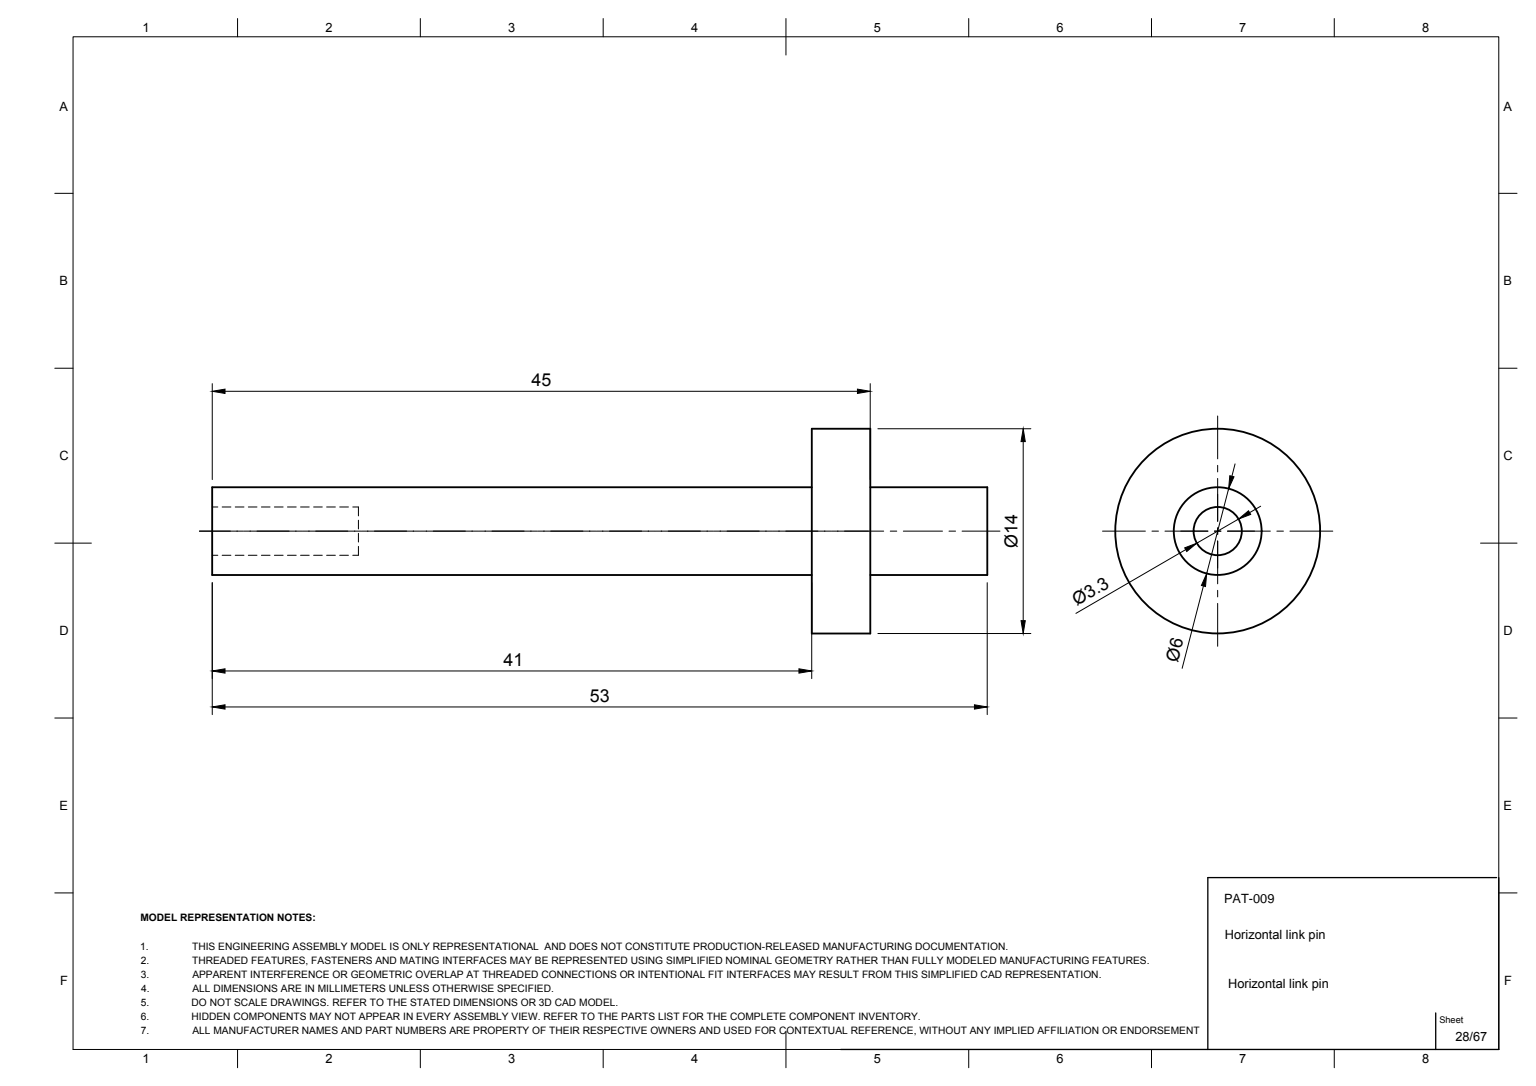
ISO-10303-21;
HEADER;
/* Generated by software containing ST-Developer
 * from STEP Tools, Inc. (www.steptools.com) 
 */

FILE_DESCRIPTION(
/* description */ ('Bell-crank linkage with push rods'),
/* implementation_level */ '2;1');

FILE_NAME(
/* name */ 'Horizontal link pin.step',
/* time_stamp */ '2026-10-28T03:25:15-07:00',
/* author */ (''),
/* organization */ (''),
/* preprocessor_version */ 'ST-DEVELOPER v20.2',
/* originating_system */ 'Autodesk Translation Framework v15.17.0.0',
/* authorisation */ '');

FILE_SCHEMA (('AUTOMOTIVE_DESIGN { 1 0 10303 214 3 1 1 }'));
ENDSEC;

DATA;
#10=MECHANICAL_DESIGN_GEOMETRIC_PRESENTATION_REPRESENTATION('',(#633),#16678);
#517=SHAPE_REPRESENTATION_RELATIONSHIP('SRR','None',#16935,#571);
#571=ADVANCED_BREP_SHAPE_REPRESENTATION('',(#694),#16640);
#633=STYLED_ITEM('',(#17291),#694);
#694=MANIFOLD_SOLID_BREP('Body1',#8824);
#838=FACE_BOUND('',#2152,.T.);
#839=FACE_BOUND('',#2154,.T.);
#840=FACE_BOUND('',#2159,.T.);
#1101=PLANE('',#10029);
#1102=PLANE('',#10030);
#1103=PLANE('',#10033);
#1104=PLANE('',#10041);
#1105=PLANE('',#10042);
#1514=FACE_OUTER_BOUND('',#2149,.T.);
#1515=FACE_OUTER_BOUND('',#2150,.T.);
#1516=FACE_OUTER_BOUND('',#2151,.T.);
#1517=FACE_OUTER_BOUND('',#2153,.T.);
#1518=FACE_OUTER_BOUND('',#2155,.T.);
#1519=FACE_OUTER_BOUND('',#2156,.T.);
#1520=FACE_OUTER_BOUND('',#2157,.T.);
#1521=FACE_OUTER_BOUND('',#2158,.T.);
#1522=FACE_OUTER_BOUND('',#2160,.T.);
#2149=EDGE_LOOP('',(#7105,#7106,#7107,#7108));
#2150=EDGE_LOOP('',(#7109));
#2151=EDGE_LOOP('',(#7110));
#2152=EDGE_LOOP('',(#7111));
#2153=EDGE_LOOP('',(#7112));
#2154=EDGE_LOOP('',(#7113));
#2155=EDGE_LOOP('',(#7114,#7115,#7116,#7117));
#2156=EDGE_LOOP('',(#7118,#7119,#7120,#7121));
#2157=EDGE_LOOP('',(#7122,#7123,#7124,#7125));
#2158=EDGE_LOOP('',(#7126));
#2159=EDGE_LOOP('',(#7127));
#2160=EDGE_LOOP('',(#7128));
#2816=LINE('',#15368,#3365);
#2817=LINE('',#15382,#3366);
#2818=LINE('',#15385,#3367);
#2819=LINE('',#15390,#3368);
#3365=VECTOR('',#12062,0.165);
#3366=VECTOR('',#12081,0.7);
#3367=VECTOR('',#12084,0.3);
#3368=VECTOR('',#12091,0.3);
#3904=CIRCLE('',#10027,0.165);
#3905=CIRCLE('',#10028,0.165);
#3906=CIRCLE('',#10031,0.7);
#3907=CIRCLE('',#10032,0.3);
#3908=CIRCLE('',#10034,0.7);
#3909=CIRCLE('',#10035,0.3);
#3910=CIRCLE('',#10038,0.3);
#3911=CIRCLE('',#10040,0.3);
#4515=VERTEX_POINT('',#15365);
#4516=VERTEX_POINT('',#15367);
#4517=VERTEX_POINT('',#15372);
#4518=VERTEX_POINT('',#15374);
#4519=VERTEX_POINT('',#15377);
#4520=VERTEX_POINT('',#15379);
#4521=VERTEX_POINT('',#15384);
#4522=VERTEX_POINT('',#15388);
#5430=EDGE_CURVE('',#4515,#4515,#3904,.T.);
#5431=EDGE_CURVE('',#4515,#4516,#2816,.T.);
#5432=EDGE_CURVE('',#4516,#4516,#3905,.T.);
#5433=EDGE_CURVE('',#4517,#4517,#3906,.T.);
#5434=EDGE_CURVE('',#4518,#4518,#3907,.T.);
#5435=EDGE_CURVE('',#4519,#4519,#3908,.T.);
#5436=EDGE_CURVE('',#4520,#4520,#3909,.T.);
#5437=EDGE_CURVE('',#4517,#4519,#2817,.T.);
#5438=EDGE_CURVE('',#4520,#4521,#2818,.T.);
#5439=EDGE_CURVE('',#4521,#4521,#3910,.T.);
#5440=EDGE_CURVE('',#4522,#4522,#3911,.T.);
#5441=EDGE_CURVE('',#4522,#4518,#2819,.T.);
#7105=ORIENTED_EDGE('',*,*,#5430,.F.);
#7106=ORIENTED_EDGE('',*,*,#5431,.T.);
#7107=ORIENTED_EDGE('',*,*,#5432,.F.);
#7108=ORIENTED_EDGE('',*,*,#5431,.F.);
#7109=ORIENTED_EDGE('',*,*,#5430,.T.);
#7110=ORIENTED_EDGE('',*,*,#5433,.T.);
#7111=ORIENTED_EDGE('',*,*,#5434,.F.);
#7112=ORIENTED_EDGE('',*,*,#5435,.F.);
#7113=ORIENTED_EDGE('',*,*,#5436,.F.);
#7114=ORIENTED_EDGE('',*,*,#5433,.F.);
#7115=ORIENTED_EDGE('',*,*,#5437,.T.);
#7116=ORIENTED_EDGE('',*,*,#5435,.T.);
#7117=ORIENTED_EDGE('',*,*,#5437,.F.);
#7118=ORIENTED_EDGE('',*,*,#5436,.T.);
#7119=ORIENTED_EDGE('',*,*,#5438,.T.);
#7120=ORIENTED_EDGE('',*,*,#5439,.T.);
#7121=ORIENTED_EDGE('',*,*,#5438,.F.);
#7122=ORIENTED_EDGE('',*,*,#5440,.F.);
#7123=ORIENTED_EDGE('',*,*,#5441,.T.);
#7124=ORIENTED_EDGE('',*,*,#5434,.T.);
#7125=ORIENTED_EDGE('',*,*,#5441,.F.);
#7126=ORIENTED_EDGE('',*,*,#5440,.T.);
#7127=ORIENTED_EDGE('',*,*,#5432,.T.);
#7128=ORIENTED_EDGE('',*,*,#5439,.F.);
#8171=CYLINDRICAL_SURFACE('',#10026,0.165);
#8172=CYLINDRICAL_SURFACE('',#10036,0.7);
#8173=CYLINDRICAL_SURFACE('',#10037,0.3);
#8174=CYLINDRICAL_SURFACE('',#10039,0.3);
#8539=ADVANCED_FACE('',(#1514),#8171,.F.);
#8540=ADVANCED_FACE('',(#1515),#1101,.T.);
#8541=ADVANCED_FACE('',(#1516,#838),#1102,.T.);
#8542=ADVANCED_FACE('',(#1517,#839),#1103,.F.);
#8543=ADVANCED_FACE('',(#1518),#8172,.T.);
#8544=ADVANCED_FACE('',(#1519),#8173,.T.);
#8545=ADVANCED_FACE('',(#1520),#8174,.T.);
#8546=ADVANCED_FACE('',(#1521,#840),#1104,.T.);
#8547=ADVANCED_FACE('',(#1522),#1105,.F.);
#8824=CLOSED_SHELL('',(#8539,#8540,#8541,#8542,#8543,#8544,#8545,#8546,
#8547));
#10025=AXIS2_PLACEMENT_3D('',#15363,#12056,#12057);
#10026=AXIS2_PLACEMENT_3D('',#15364,#12058,#12059);
#10027=AXIS2_PLACEMENT_3D('',#15366,#12060,#12061);
#10028=AXIS2_PLACEMENT_3D('',#15369,#12063,#12064);
#10029=AXIS2_PLACEMENT_3D('',#15370,#12065,#12066);
#10030=AXIS2_PLACEMENT_3D('',#15371,#12067,#12068);
#10031=AXIS2_PLACEMENT_3D('',#15373,#12069,#12070);
#10032=AXIS2_PLACEMENT_3D('',#15375,#12071,#12072);
#10033=AXIS2_PLACEMENT_3D('',#15376,#12073,#12074);
#10034=AXIS2_PLACEMENT_3D('',#15378,#12075,#12076);
#10035=AXIS2_PLACEMENT_3D('',#15380,#12077,#12078);
#10036=AXIS2_PLACEMENT_3D('',#15381,#12079,#12080);
#10037=AXIS2_PLACEMENT_3D('',#15383,#12082,#12083);
#10038=AXIS2_PLACEMENT_3D('',#15386,#12085,#12086);
#10039=AXIS2_PLACEMENT_3D('',#15387,#12087,#12088);
#10040=AXIS2_PLACEMENT_3D('',#15389,#12089,#12090);
#10041=AXIS2_PLACEMENT_3D('',#15391,#12092,#12093);
#10042=AXIS2_PLACEMENT_3D('',#15392,#12094,#12095);
#12056=DIRECTION('axis',(0.,0.,1.));
#12057=DIRECTION('refdir',(1.,0.,0.));
#12058=DIRECTION('center_axis',(0.,0.,1.));
#12059=DIRECTION('ref_axis',(1.,0.,0.));
#12060=DIRECTION('center_axis',(0.,0.,1.));
#12061=DIRECTION('ref_axis',(1.,0.,0.));
#12062=DIRECTION('',(0.,0.,1.));
#12063=DIRECTION('center_axis',(0.,0.,-1.));
#12064=DIRECTION('ref_axis',(1.,0.,0.));
#12065=DIRECTION('center_axis',(0.,0.,1.));
#12066=DIRECTION('ref_axis',(1.,0.,0.));
#12067=DIRECTION('center_axis',(0.,0.,1.));
#12068=DIRECTION('ref_axis',(1.,0.,0.));
#12069=DIRECTION('center_axis',(0.,0.,1.));
#12070=DIRECTION('ref_axis',(1.,0.,0.));
#12071=DIRECTION('center_axis',(0.,0.,1.));
#12072=DIRECTION('ref_axis',(1.,0.,0.));
#12073=DIRECTION('center_axis',(0.,0.,1.));
#12074=DIRECTION('ref_axis',(1.,0.,0.));
#12075=DIRECTION('center_axis',(0.,0.,1.));
#12076=DIRECTION('ref_axis',(1.,0.,0.));
#12077=DIRECTION('center_axis',(0.,0.,-1.));
#12078=DIRECTION('ref_axis',(1.,0.,0.));
#12079=DIRECTION('center_axis',(0.,0.,1.));
#12080=DIRECTION('ref_axis',(1.,0.,0.));
#12081=DIRECTION('',(0.,0.,-1.));
#12082=DIRECTION('center_axis',(0.,0.,1.));
#12083=DIRECTION('ref_axis',(1.,0.,0.));
#12084=DIRECTION('',(0.,0.,-1.));
#12085=DIRECTION('center_axis',(0.,0.,1.));
#12086=DIRECTION('ref_axis',(1.,0.,0.));
#12087=DIRECTION('center_axis',(0.,0.,1.));
#12088=DIRECTION('ref_axis',(1.,0.,0.));
#12089=DIRECTION('center_axis',(0.,0.,1.));
#12090=DIRECTION('ref_axis',(1.,0.,0.));
#12091=DIRECTION('',(0.,0.,-1.));
#12092=DIRECTION('center_axis',(0.,0.,1.));
#12093=DIRECTION('ref_axis',(1.,0.,0.));
#12094=DIRECTION('center_axis',(0.,0.,1.));
#12095=DIRECTION('ref_axis',(1.,0.,0.));
#15363=CARTESIAN_POINT('',(0.,0.,0.));
#15364=CARTESIAN_POINT('Origin',(0.,2.,9.1));
#15365=CARTESIAN_POINT('',(-0.165,2.,9.1));
#15366=CARTESIAN_POINT('Origin',(0.,2.,9.1));
#15367=CARTESIAN_POINT('',(-0.165,2.,10.1));
#15368=CARTESIAN_POINT('',(-0.165,2.,9.1));
#15369=CARTESIAN_POINT('Origin',(0.,2.,10.1));
#15370=CARTESIAN_POINT('Origin',(0.,2.,9.1));
#15371=CARTESIAN_POINT('Origin',(0.,2.,6.));
#15372=CARTESIAN_POINT('',(-0.7,2.,6.));
#15373=CARTESIAN_POINT('Origin',(0.,2.,6.));
#15374=CARTESIAN_POINT('',(-0.3,2.,6.));
#15375=CARTESIAN_POINT('Origin',(0.,2.,6.));
#15376=CARTESIAN_POINT('Origin',(0.,2.,5.6));
#15377=CARTESIAN_POINT('',(-0.7,2.,5.6));
#15378=CARTESIAN_POINT('Origin',(0.,2.,5.6));
#15379=CARTESIAN_POINT('',(-0.3,2.,5.6));
#15380=CARTESIAN_POINT('Origin',(0.,2.,5.6));
#15381=CARTESIAN_POINT('Origin',(0.,2.,5.6));
#15382=CARTESIAN_POINT('',(-0.7,2.,5.6));
#15383=CARTESIAN_POINT('Origin',(0.,2.,4.8));
#15384=CARTESIAN_POINT('',(-0.3,2.,4.8));
#15385=CARTESIAN_POINT('',(-0.3,2.,4.8));
#15386=CARTESIAN_POINT('Origin',(0.,2.,4.8));
#15387=CARTESIAN_POINT('Origin',(0.,2.,4.8));
#15388=CARTESIAN_POINT('',(-0.3,2.,10.1));
#15389=CARTESIAN_POINT('Origin',(0.,2.,10.1));
#15390=CARTESIAN_POINT('',(-0.3,2.,4.8));
#15391=CARTESIAN_POINT('Origin',(0.,2.,10.1));
#15392=CARTESIAN_POINT('Origin',(0.,2.,4.8));
#16576=UNCERTAINTY_MEASURE_WITH_UNIT(LENGTH_MEASURE(0.001),#16679,
'DISTANCE_ACCURACY_VALUE',
'Maximum model space distance between geometric entities at asserted c
onnectivities');
#16614=UNCERTAINTY_MEASURE_WITH_UNIT(LENGTH_MEASURE(0.001),#16679,
'DISTANCE_ACCURACY_VALUE',
'Maximum model space distance between geometric entities at asserted c
onnectivities');
#16640=(
GEOMETRIC_REPRESENTATION_CONTEXT(3)
GLOBAL_UNCERTAINTY_ASSIGNED_CONTEXT((#16576))
GLOBAL_UNIT_ASSIGNED_CONTEXT((#16679,#16681,#16682))
REPRESENTATION_CONTEXT('','3D')
);
#16678=(
GEOMETRIC_REPRESENTATION_CONTEXT(3)
GLOBAL_UNCERTAINTY_ASSIGNED_CONTEXT((#16614))
GLOBAL_UNIT_ASSIGNED_CONTEXT((#16679,#16681,#16682))
REPRESENTATION_CONTEXT('','3D')
);
#16679=(
LENGTH_UNIT()
NAMED_UNIT(*)
SI_UNIT(.CENTI.,.METRE.)
);
#16681=(
NAMED_UNIT(*)
PLANE_ANGLE_UNIT()
SI_UNIT($,.RADIAN.)
);
#16682=(
NAMED_UNIT(*)
SI_UNIT($,.STERADIAN.)
SOLID_ANGLE_UNIT()
);
#16708=SHAPE_DEFINITION_REPRESENTATION(#16776,#16935);
#16776=PRODUCT_DEFINITION_SHAPE('',$,#16999);
#16935=SHAPE_REPRESENTATION('',(#10025),#16640);
#16973=PRODUCT_DEFINITION_CONTEXT('part definition',#17164,'design');
#16999=PRODUCT_DEFINITION('Horizontal link pin','Horizontal link pin',#17062,
#16973);
#17062=PRODUCT_DEFINITION_FORMATION('',$,#17191);
#17164=APPLICATION_CONTEXT(
'Core Data for Automotive Mechanical Design Process');
#17165=PRODUCT_CONTEXT('part definition',#17164,'mechanical');
#17191=PRODUCT('Horizontal link pin','Horizontal link pin',
'Horizontal link pin',(#17165));
#17285=COLOUR_RGB('Grey',0.48,0.52,0.57);
#17286=FILL_AREA_STYLE_COLOUR('',#17285);
#17287=FILL_AREA_STYLE('',(#17286));
#17288=SURFACE_STYLE_FILL_AREA(#17287);
#17289=SURFACE_SIDE_STYLE('',(#17288));
#17290=SURFACE_STYLE_USAGE(.BOTH.,#17289);
#17291=PRESENTATION_STYLE_ASSIGNMENT((#17290));
ENDSEC;
END-ISO-10303-21;
